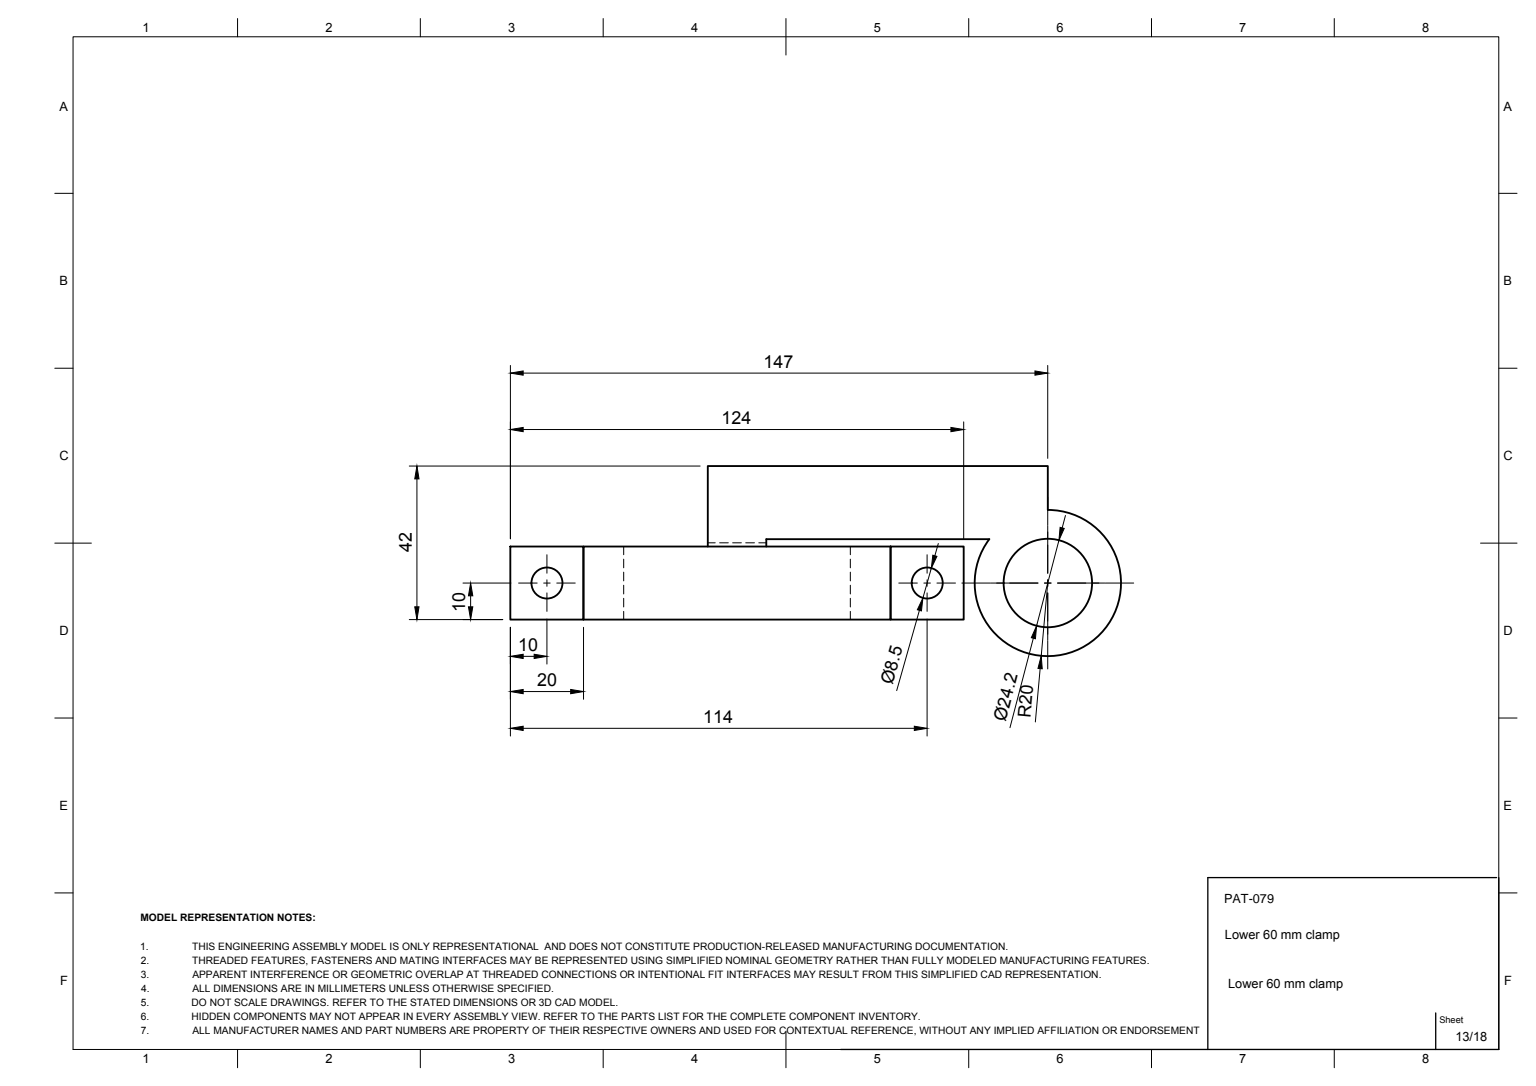
ISO-10303-21;
HEADER;
/* Generated by software containing ST-Developer
 * from STEP Tools, Inc. (www.steptools.com) 
 */

FILE_DESCRIPTION(
/* description */ ('Pipe clamp stand with threaded column'),
/* implementation_level */ '2;1');

FILE_NAME(
/* name */ 'Lower 60 mm clamp.step',
/* time_stamp */ '2026-10-27T10:55:48-07:00',
/* author */ (''),
/* organization */ (''),
/* preprocessor_version */ 'ST-DEVELOPER v20.2',
/* originating_system */ 'Autodesk Translation Framework v15.17.0.0',
/* authorisation */ '');

FILE_SCHEMA (('AUTOMOTIVE_DESIGN { 1 0 10303 214 3 1 1 }'));
ENDSEC;

DATA;
#10=MECHANICAL_DESIGN_GEOMETRIC_PRESENTATION_REPRESENTATION('',(#753,#754,#755),#34433);
#705=SHAPE_REPRESENTATION_RELATIONSHIP('SRR','None',#34547,#727);
#727=ADVANCED_BREP_SHAPE_REPRESENTATION('',(#783,#784,#785),#34415);
#753=STYLED_ITEM('',(#34757),#783);
#754=STYLED_ITEM('',(#34757),#784);
#755=STYLED_ITEM('',(#34757),#785);
#783=MANIFOLD_SOLID_BREP('Body1',#8780);
#784=MANIFOLD_SOLID_BREP('Body2',#8781);
#785=MANIFOLD_SOLID_BREP('Body3',#8782);
#832=FACE_BOUND('',#1857,.T.);
#833=FACE_BOUND('',#1861,.T.);
#834=FACE_BOUND('',#1869,.T.);
#835=FACE_BOUND('',#1872,.T.);
#836=FACE_BOUND('',#1878,.T.);
#837=FACE_BOUND('',#1881,.T.);
#919=PLANE('',#9405);
#920=PLANE('',#9406);
#921=PLANE('',#9408);
#922=PLANE('',#9409);
#923=PLANE('',#9416);
#924=PLANE('',#9417);
#925=PLANE('',#9418);
#926=PLANE('',#9419);
#927=PLANE('',#9420);
#928=PLANE('',#9421);
#929=PLANE('',#9422);
#930=PLANE('',#9423);
#931=PLANE('',#9429);
#932=PLANE('',#9430);
#933=PLANE('',#9431);
#934=PLANE('',#9432);
#935=PLANE('',#9433);
#936=PLANE('',#9434);
#937=PLANE('',#9438);
#938=PLANE('',#9439);
#939=PLANE('',#9440);
#940=PLANE('',#9441);
#941=PLANE('',#9442);
#942=PLANE('',#9443);
#1328=FACE_OUTER_BOUND('',#1848,.T.);
#1329=FACE_OUTER_BOUND('',#1849,.T.);
#1330=FACE_OUTER_BOUND('',#1850,.T.);
#1331=FACE_OUTER_BOUND('',#1851,.T.);
#1332=FACE_OUTER_BOUND('',#1852,.T.);
#1333=FACE_OUTER_BOUND('',#1853,.T.);
#1334=FACE_OUTER_BOUND('',#1854,.T.);
#1335=FACE_OUTER_BOUND('',#1855,.T.);
#1336=FACE_OUTER_BOUND('',#1856,.T.);
#1337=FACE_OUTER_BOUND('',#1858,.T.);
#1338=FACE_OUTER_BOUND('',#1859,.T.);
#1339=FACE_OUTER_BOUND('',#1860,.T.);
#1340=FACE_OUTER_BOUND('',#1862,.T.);
#1341=FACE_OUTER_BOUND('',#1863,.T.);
#1342=FACE_OUTER_BOUND('',#1864,.T.);
#1343=FACE_OUTER_BOUND('',#1865,.T.);
#1344=FACE_OUTER_BOUND('',#1866,.T.);
#1345=FACE_OUTER_BOUND('',#1867,.T.);
#1346=FACE_OUTER_BOUND('',#1868,.T.);
#1347=FACE_OUTER_BOUND('',#1870,.T.);
#1348=FACE_OUTER_BOUND('',#1871,.T.);
#1349=FACE_OUTER_BOUND('',#1873,.T.);
#1350=FACE_OUTER_BOUND('',#1874,.T.);
#1351=FACE_OUTER_BOUND('',#1875,.T.);
#1352=FACE_OUTER_BOUND('',#1876,.T.);
#1353=FACE_OUTER_BOUND('',#1877,.T.);
#1354=FACE_OUTER_BOUND('',#1879,.T.);
#1355=FACE_OUTER_BOUND('',#1880,.T.);
#1356=FACE_OUTER_BOUND('',#1882,.T.);
#1357=FACE_OUTER_BOUND('',#1883,.T.);
#1848=EDGE_LOOP('',(#7055,#7056,#7057,#7058,#7059,#7060,#7061,#7062));
#1849=EDGE_LOOP('',(#7063,#7064,#7065,#7066));
#1850=EDGE_LOOP('',(#7067,#7068,#7069,#7070));
#1851=EDGE_LOOP('',(#7071,#7072,#7073,#7074));
#1852=EDGE_LOOP('',(#7075,#7076,#7077,#7078,#7079,#7080));
#1853=EDGE_LOOP('',(#7081,#7082,#7083,#7084));
#1854=EDGE_LOOP('',(#7085,#7086,#7087,#7088));
#1855=EDGE_LOOP('',(#7089,#7090,#7091,#7092));
#1856=EDGE_LOOP('',(#7093,#7094,#7095,#7096,#7097,#7098,#7099));
#1857=EDGE_LOOP('',(#7100));
#1858=EDGE_LOOP('',(#7101,#7102,#7103,#7104));
#1859=EDGE_LOOP('',(#7105,#7106,#7107,#7108));
#1860=EDGE_LOOP('',(#7109,#7110,#7111,#7112,#7113,#7114,#7115));
#1861=EDGE_LOOP('',(#7116));
#1862=EDGE_LOOP('',(#7117,#7118,#7119,#7120,#7121,#7122));
#1863=EDGE_LOOP('',(#7123,#7124,#7125,#7126));
#1864=EDGE_LOOP('',(#7127,#7128,#7129,#7130,#7131,#7132,#7133,#7134));
#1865=EDGE_LOOP('',(#7135,#7136,#7137,#7138));
#1866=EDGE_LOOP('',(#7139,#7140,#7141,#7142));
#1867=EDGE_LOOP('',(#7143,#7144,#7145,#7146));
#1868=EDGE_LOOP('',(#7147,#7148,#7149,#7150));
#1869=EDGE_LOOP('',(#7151));
#1870=EDGE_LOOP('',(#7152,#7153,#7154,#7155));
#1871=EDGE_LOOP('',(#7156,#7157,#7158,#7159));
#1872=EDGE_LOOP('',(#7160));
#1873=EDGE_LOOP('',(#7161,#7162,#7163,#7164));
#1874=EDGE_LOOP('',(#7165,#7166,#7167,#7168));
#1875=EDGE_LOOP('',(#7169,#7170,#7171,#7172));
#1876=EDGE_LOOP('',(#7173,#7174,#7175,#7176));
#1877=EDGE_LOOP('',(#7177,#7178,#7179,#7180));
#1878=EDGE_LOOP('',(#7181));
#1879=EDGE_LOOP('',(#7182,#7183,#7184,#7185));
#1880=EDGE_LOOP('',(#7186,#7187,#7188,#7189));
#1881=EDGE_LOOP('',(#7190));
#1882=EDGE_LOOP('',(#7191,#7192,#7193,#7194));
#1883=EDGE_LOOP('',(#7195,#7196,#7197,#7198));
#2399=LINE('',#28332,#3016);
#2400=LINE('',#28336,#3017);
#2401=LINE('',#28340,#3018);
#2402=LINE('',#28344,#3019);
#2403=LINE('',#28348,#3020);
#2404=LINE('',#28350,#3021);
#2405=LINE('',#28351,#3022);
#2406=LINE('',#28354,#3023);
#2407=LINE('',#28357,#3024);
#2408=LINE('',#28360,#3025);
#2409=LINE('',#28361,#3026);
#2410=LINE('',#28364,#3027);
#2411=LINE('',#28366,#3028);
#2412=LINE('',#28368,#3029);
#2413=LINE('',#28369,#3030);
#2414=LINE('',#28374,#3031);
#2415=LINE('',#28379,#3032);
#2416=LINE('',#28383,#3033);
#2417=LINE('',#28386,#3034);
#2418=LINE('',#28387,#3035);
#2419=LINE('',#28390,#3036);
#2420=LINE('',#28392,#3037);
#2421=LINE('',#28394,#3038);
#2422=LINE('',#28395,#3039);
#2423=LINE('',#28398,#3040);
#2424=LINE('',#28399,#3041);
#2425=LINE('',#28402,#3042);
#2426=LINE('',#28403,#3043);
#2427=LINE('',#28405,#3044);
#2428=LINE('',#28407,#3045);
#2429=LINE('',#28410,#3046);
#2430=LINE('',#28411,#3047);
#2431=LINE('',#28419,#3048);
#2432=LINE('',#28424,#3049);
#2433=LINE('',#28426,#3050);
#2434=LINE('',#28428,#3051);
#2435=LINE('',#28429,#3052);
#2436=LINE('',#28432,#3053);
#2437=LINE('',#28434,#3054);
#2438=LINE('',#28435,#3055);
#2439=LINE('',#28438,#3056);
#2440=LINE('',#28440,#3057);
#2441=LINE('',#28441,#3058);
#2442=LINE('',#28443,#3059);
#2443=LINE('',#28444,#3060);
#2444=LINE('',#28451,#3061);
#2445=LINE('',#28456,#3062);
#2446=LINE('',#28458,#3063);
#2447=LINE('',#28460,#3064);
#2448=LINE('',#28461,#3065);
#2449=LINE('',#28464,#3066);
#2450=LINE('',#28466,#3067);
#2451=LINE('',#28467,#3068);
#2452=LINE('',#28470,#3069);
#2453=LINE('',#28472,#3070);
#2454=LINE('',#28473,#3071);
#2455=LINE('',#28475,#3072);
#2456=LINE('',#28476,#3073);
#3016=VECTOR('',#10764,1.);
#3017=VECTOR('',#10767,1.);
#3018=VECTOR('',#10770,1.);
#3019=VECTOR('',#10773,1.);
#3020=VECTOR('',#10778,1.);
#3021=VECTOR('',#10779,1.);
#3022=VECTOR('',#10780,1.);
#3023=VECTOR('',#10783,1.);
#3024=VECTOR('',#10786,1.);
#3025=VECTOR('',#10789,1.);
#3026=VECTOR('',#10790,1.);
#3027=VECTOR('',#10793,1.);
#3028=VECTOR('',#10794,1.);
#3029=VECTOR('',#10795,1.);
#3030=VECTOR('',#10796,1.);
#3031=VECTOR('',#10801,1.21);
#3032=VECTOR('',#10806,1.);
#3033=VECTOR('',#10809,1.);
#3034=VECTOR('',#10814,1.);
#3035=VECTOR('',#10815,1.);
#3036=VECTOR('',#10818,1.);
#3037=VECTOR('',#10819,1.);
#3038=VECTOR('',#10820,1.);
#3039=VECTOR('',#10821,1.);
#3040=VECTOR('',#10824,1.);
#3041=VECTOR('',#10825,1.);
#3042=VECTOR('',#10828,1.);
#3043=VECTOR('',#10829,1.);
#3044=VECTOR('',#10832,1.);
#3045=VECTOR('',#10835,1.);
#3046=VECTOR('',#10838,1.);
#3047=VECTOR('',#10839,1.);
#3048=VECTOR('',#10850,0.425);
#3049=VECTOR('',#10855,1.);
#3050=VECTOR('',#10856,1.);
#3051=VECTOR('',#10857,1.);
#3052=VECTOR('',#10858,1.);
#3053=VECTOR('',#10861,1.);
#3054=VECTOR('',#10862,1.);
#3055=VECTOR('',#10863,1.);
#3056=VECTOR('',#10866,1.);
#3057=VECTOR('',#10867,1.);
#3058=VECTOR('',#10868,1.);
#3059=VECTOR('',#10871,1.);
#3060=VECTOR('',#10872,1.);
#3061=VECTOR('',#10881,0.425);
#3062=VECTOR('',#10886,1.);
#3063=VECTOR('',#10887,1.);
#3064=VECTOR('',#10888,1.);
#3065=VECTOR('',#10889,1.);
#3066=VECTOR('',#10892,1.);
#3067=VECTOR('',#10893,1.);
#3068=VECTOR('',#10894,1.);
#3069=VECTOR('',#10897,1.);
#3070=VECTOR('',#10898,1.);
#3071=VECTOR('',#10899,1.);
#3072=VECTOR('',#10902,1.);
#3073=VECTOR('',#10903,1.);
#3374=CIRCLE('',#9401,3.1);
#3375=CIRCLE('',#9402,3.1);
#3376=CIRCLE('',#9403,3.1);
#3377=CIRCLE('',#9404,3.1);
#3378=CIRCLE('',#9407,4.2);
#3379=CIRCLE('',#9411,1.21);
#3380=CIRCLE('',#9412,1.21);
#3381=CIRCLE('',#9414,2.);
#3382=CIRCLE('',#9415,2.);
#3383=CIRCLE('',#9424,4.2);
#3384=CIRCLE('',#9427,0.425);
#3385=CIRCLE('',#9428,0.425);
#3386=CIRCLE('',#9436,0.425);
#3387=CIRCLE('',#9437,0.425);
#3958=VERTEX_POINT('',#28330);
#3959=VERTEX_POINT('',#28331);
#3960=VERTEX_POINT('',#28333);
#3961=VERTEX_POINT('',#28335);
#3962=VERTEX_POINT('',#28337);
#3963=VERTEX_POINT('',#28339);
#3964=VERTEX_POINT('',#28341);
#3965=VERTEX_POINT('',#28343);
#3966=VERTEX_POINT('',#28347);
#3967=VERTEX_POINT('',#28349);
#3968=VERTEX_POINT('',#28353);
#3969=VERTEX_POINT('',#28355);
#3970=VERTEX_POINT('',#28359);
#3971=VERTEX_POINT('',#28363);
#3972=VERTEX_POINT('',#28365);
#3973=VERTEX_POINT('',#28367);
#3974=VERTEX_POINT('',#28371);
#3975=VERTEX_POINT('',#28373);
#3976=VERTEX_POINT('',#28377);
#3977=VERTEX_POINT('',#28378);
#3978=VERTEX_POINT('',#28380);
#3979=VERTEX_POINT('',#28382);
#3980=VERTEX_POINT('',#28389);
#3981=VERTEX_POINT('',#28391);
#3982=VERTEX_POINT('',#28393);
#3983=VERTEX_POINT('',#28397);
#3984=VERTEX_POINT('',#28401);
#3985=VERTEX_POINT('',#28409);
#3986=VERTEX_POINT('',#28416);
#3987=VERTEX_POINT('',#28418);
#3988=VERTEX_POINT('',#28422);
#3989=VERTEX_POINT('',#28423);
#3990=VERTEX_POINT('',#28425);
#3991=VERTEX_POINT('',#28427);
#3992=VERTEX_POINT('',#28431);
#3993=VERTEX_POINT('',#28433);
#3994=VERTEX_POINT('',#28437);
#3995=VERTEX_POINT('',#28439);
#3996=VERTEX_POINT('',#28448);
#3997=VERTEX_POINT('',#28450);
#3998=VERTEX_POINT('',#28454);
#3999=VERTEX_POINT('',#28455);
#4000=VERTEX_POINT('',#28457);
#4001=VERTEX_POINT('',#28459);
#4002=VERTEX_POINT('',#28463);
#4003=VERTEX_POINT('',#28465);
#4004=VERTEX_POINT('',#28469);
#4005=VERTEX_POINT('',#28471);
#5041=EDGE_CURVE('',#3958,#3959,#2399,.T.);
#5042=EDGE_CURVE('',#3958,#3960,#3374,.T.);
#5043=EDGE_CURVE('',#3961,#3960,#2400,.T.);
#5044=EDGE_CURVE('',#3962,#3961,#3375,.T.);
#5045=EDGE_CURVE('',#3963,#3962,#2401,.T.);
#5046=EDGE_CURVE('',#3964,#3963,#3376,.T.);
#5047=EDGE_CURVE('',#3965,#3964,#2402,.T.);
#5048=EDGE_CURVE('',#3959,#3965,#3377,.T.);
#5049=EDGE_CURVE('',#3966,#3958,#2403,.T.);
#5050=EDGE_CURVE('',#3967,#3966,#2404,.T.);
#5051=EDGE_CURVE('',#3960,#3967,#2405,.T.);
#5052=EDGE_CURVE('',#3963,#3968,#2406,.T.);
#5053=EDGE_CURVE('',#3969,#3968,#3378,.T.);
#5054=EDGE_CURVE('',#3969,#3964,#2407,.T.);
#5055=EDGE_CURVE('',#3970,#3962,#2408,.T.);
#5056=EDGE_CURVE('',#3968,#3970,#2409,.T.);
#5057=EDGE_CURVE('',#3967,#3971,#2410,.T.);
#5058=EDGE_CURVE('',#3971,#3972,#2411,.T.);
#5059=EDGE_CURVE('',#3973,#3972,#2412,.T.);
#5060=EDGE_CURVE('',#3961,#3973,#2413,.T.);
#5061=EDGE_CURVE('',#3974,#3974,#3379,.T.);
#5062=EDGE_CURVE('',#3974,#3975,#2414,.T.);
#5063=EDGE_CURVE('',#3975,#3975,#3380,.T.);
#5064=EDGE_CURVE('',#3976,#3977,#2415,.T.);
#5065=EDGE_CURVE('',#3978,#3976,#3381,.T.);
#5066=EDGE_CURVE('',#3979,#3978,#2416,.T.);
#5067=EDGE_CURVE('',#3979,#3977,#3382,.T.);
#5068=EDGE_CURVE('',#3977,#3972,#2417,.T.);
#5069=EDGE_CURVE('',#3971,#3976,#2418,.T.);
#5070=EDGE_CURVE('',#3979,#3980,#2419,.T.);
#5071=EDGE_CURVE('',#3981,#3980,#2420,.T.);
#5072=EDGE_CURVE('',#3982,#3981,#2421,.T.);
#5073=EDGE_CURVE('',#3973,#3982,#2422,.T.);
#5074=EDGE_CURVE('',#3978,#3983,#2423,.T.);
#5075=EDGE_CURVE('',#3980,#3983,#2424,.T.);
#5076=EDGE_CURVE('',#3983,#3984,#2425,.T.);
#5077=EDGE_CURVE('',#3984,#3981,#2426,.T.);
#5078=EDGE_CURVE('',#3966,#3984,#2427,.T.);
#5079=EDGE_CURVE('',#3982,#3959,#2428,.T.);
#5080=EDGE_CURVE('',#3985,#3969,#2429,.T.);
#5081=EDGE_CURVE('',#3965,#3985,#2430,.T.);
#5082=EDGE_CURVE('',#3985,#3970,#3383,.T.);
#5083=EDGE_CURVE('',#3986,#3986,#3384,.T.);
#5084=EDGE_CURVE('',#3986,#3987,#2431,.T.);
#5085=EDGE_CURVE('',#3987,#3987,#3385,.T.);
#5086=EDGE_CURVE('',#3988,#3989,#2432,.T.);
#5087=EDGE_CURVE('',#3988,#3990,#2433,.T.);
#5088=EDGE_CURVE('',#3991,#3990,#2434,.T.);
#5089=EDGE_CURVE('',#3989,#3991,#2435,.T.);
#5090=EDGE_CURVE('',#3989,#3992,#2436,.T.);
#5091=EDGE_CURVE('',#3993,#3991,#2437,.T.);
#5092=EDGE_CURVE('',#3992,#3993,#2438,.T.);
#5093=EDGE_CURVE('',#3992,#3994,#2439,.T.);
#5094=EDGE_CURVE('',#3995,#3993,#2440,.T.);
#5095=EDGE_CURVE('',#3994,#3995,#2441,.T.);
#5096=EDGE_CURVE('',#3994,#3988,#2442,.T.);
#5097=EDGE_CURVE('',#3990,#3995,#2443,.T.);
#5098=EDGE_CURVE('',#3996,#3996,#3386,.T.);
#5099=EDGE_CURVE('',#3996,#3997,#2444,.T.);
#5100=EDGE_CURVE('',#3997,#3997,#3387,.T.);
#5101=EDGE_CURVE('',#3998,#3999,#2445,.T.);
#5102=EDGE_CURVE('',#3998,#4000,#2446,.T.);
#5103=EDGE_CURVE('',#4001,#4000,#2447,.T.);
#5104=EDGE_CURVE('',#3999,#4001,#2448,.T.);
#5105=EDGE_CURVE('',#3999,#4002,#2449,.T.);
#5106=EDGE_CURVE('',#4003,#4001,#2450,.T.);
#5107=EDGE_CURVE('',#4002,#4003,#2451,.T.);
#5108=EDGE_CURVE('',#4002,#4004,#2452,.T.);
#5109=EDGE_CURVE('',#4005,#4003,#2453,.T.);
#5110=EDGE_CURVE('',#4004,#4005,#2454,.T.);
#5111=EDGE_CURVE('',#4004,#3998,#2455,.T.);
#5112=EDGE_CURVE('',#4000,#4005,#2456,.T.);
#7055=ORIENTED_EDGE('',*,*,#5041,.F.);
#7056=ORIENTED_EDGE('',*,*,#5042,.T.);
#7057=ORIENTED_EDGE('',*,*,#5043,.F.);
#7058=ORIENTED_EDGE('',*,*,#5044,.F.);
#7059=ORIENTED_EDGE('',*,*,#5045,.F.);
#7060=ORIENTED_EDGE('',*,*,#5046,.F.);
#7061=ORIENTED_EDGE('',*,*,#5047,.F.);
#7062=ORIENTED_EDGE('',*,*,#5048,.F.);
#7063=ORIENTED_EDGE('',*,*,#5049,.F.);
#7064=ORIENTED_EDGE('',*,*,#5050,.F.);
#7065=ORIENTED_EDGE('',*,*,#5051,.F.);
#7066=ORIENTED_EDGE('',*,*,#5042,.F.);
#7067=ORIENTED_EDGE('',*,*,#5046,.T.);
#7068=ORIENTED_EDGE('',*,*,#5052,.T.);
#7069=ORIENTED_EDGE('',*,*,#5053,.F.);
#7070=ORIENTED_EDGE('',*,*,#5054,.T.);
#7071=ORIENTED_EDGE('',*,*,#5045,.T.);
#7072=ORIENTED_EDGE('',*,*,#5055,.F.);
#7073=ORIENTED_EDGE('',*,*,#5056,.F.);
#7074=ORIENTED_EDGE('',*,*,#5052,.F.);
#7075=ORIENTED_EDGE('',*,*,#5043,.T.);
#7076=ORIENTED_EDGE('',*,*,#5051,.T.);
#7077=ORIENTED_EDGE('',*,*,#5057,.T.);
#7078=ORIENTED_EDGE('',*,*,#5058,.T.);
#7079=ORIENTED_EDGE('',*,*,#5059,.F.);
#7080=ORIENTED_EDGE('',*,*,#5060,.F.);
#7081=ORIENTED_EDGE('',*,*,#5061,.F.);
#7082=ORIENTED_EDGE('',*,*,#5062,.T.);
#7083=ORIENTED_EDGE('',*,*,#5063,.F.);
#7084=ORIENTED_EDGE('',*,*,#5062,.F.);
#7085=ORIENTED_EDGE('',*,*,#5064,.F.);
#7086=ORIENTED_EDGE('',*,*,#5065,.F.);
#7087=ORIENTED_EDGE('',*,*,#5066,.F.);
#7088=ORIENTED_EDGE('',*,*,#5067,.T.);
#7089=ORIENTED_EDGE('',*,*,#5064,.T.);
#7090=ORIENTED_EDGE('',*,*,#5068,.T.);
#7091=ORIENTED_EDGE('',*,*,#5058,.F.);
#7092=ORIENTED_EDGE('',*,*,#5069,.T.);
#7093=ORIENTED_EDGE('',*,*,#5070,.T.);
#7094=ORIENTED_EDGE('',*,*,#5071,.F.);
#7095=ORIENTED_EDGE('',*,*,#5072,.F.);
#7096=ORIENTED_EDGE('',*,*,#5073,.F.);
#7097=ORIENTED_EDGE('',*,*,#5059,.T.);
#7098=ORIENTED_EDGE('',*,*,#5068,.F.);
#7099=ORIENTED_EDGE('',*,*,#5067,.F.);
#7100=ORIENTED_EDGE('',*,*,#5061,.T.);
#7101=ORIENTED_EDGE('',*,*,#5066,.T.);
#7102=ORIENTED_EDGE('',*,*,#5074,.T.);
#7103=ORIENTED_EDGE('',*,*,#5075,.F.);
#7104=ORIENTED_EDGE('',*,*,#5070,.F.);
#7105=ORIENTED_EDGE('',*,*,#5076,.T.);
#7106=ORIENTED_EDGE('',*,*,#5077,.T.);
#7107=ORIENTED_EDGE('',*,*,#5071,.T.);
#7108=ORIENTED_EDGE('',*,*,#5075,.T.);
#7109=ORIENTED_EDGE('',*,*,#5050,.T.);
#7110=ORIENTED_EDGE('',*,*,#5078,.T.);
#7111=ORIENTED_EDGE('',*,*,#5076,.F.);
#7112=ORIENTED_EDGE('',*,*,#5074,.F.);
#7113=ORIENTED_EDGE('',*,*,#5065,.T.);
#7114=ORIENTED_EDGE('',*,*,#5069,.F.);
#7115=ORIENTED_EDGE('',*,*,#5057,.F.);
#7116=ORIENTED_EDGE('',*,*,#5063,.T.);
#7117=ORIENTED_EDGE('',*,*,#5041,.T.);
#7118=ORIENTED_EDGE('',*,*,#5079,.F.);
#7119=ORIENTED_EDGE('',*,*,#5072,.T.);
#7120=ORIENTED_EDGE('',*,*,#5077,.F.);
#7121=ORIENTED_EDGE('',*,*,#5078,.F.);
#7122=ORIENTED_EDGE('',*,*,#5049,.T.);
#7123=ORIENTED_EDGE('',*,*,#5047,.T.);
#7124=ORIENTED_EDGE('',*,*,#5054,.F.);
#7125=ORIENTED_EDGE('',*,*,#5080,.F.);
#7126=ORIENTED_EDGE('',*,*,#5081,.F.);
#7127=ORIENTED_EDGE('',*,*,#5048,.T.);
#7128=ORIENTED_EDGE('',*,*,#5081,.T.);
#7129=ORIENTED_EDGE('',*,*,#5082,.T.);
#7130=ORIENTED_EDGE('',*,*,#5055,.T.);
#7131=ORIENTED_EDGE('',*,*,#5044,.T.);
#7132=ORIENTED_EDGE('',*,*,#5060,.T.);
#7133=ORIENTED_EDGE('',*,*,#5073,.T.);
#7134=ORIENTED_EDGE('',*,*,#5079,.T.);
#7135=ORIENTED_EDGE('',*,*,#5056,.T.);
#7136=ORIENTED_EDGE('',*,*,#5082,.F.);
#7137=ORIENTED_EDGE('',*,*,#5080,.T.);
#7138=ORIENTED_EDGE('',*,*,#5053,.T.);
#7139=ORIENTED_EDGE('',*,*,#5083,.F.);
#7140=ORIENTED_EDGE('',*,*,#5084,.T.);
#7141=ORIENTED_EDGE('',*,*,#5085,.F.);
#7142=ORIENTED_EDGE('',*,*,#5084,.F.);
#7143=ORIENTED_EDGE('',*,*,#5086,.F.);
#7144=ORIENTED_EDGE('',*,*,#5087,.T.);
#7145=ORIENTED_EDGE('',*,*,#5088,.F.);
#7146=ORIENTED_EDGE('',*,*,#5089,.F.);
#7147=ORIENTED_EDGE('',*,*,#5090,.F.);
#7148=ORIENTED_EDGE('',*,*,#5089,.T.);
#7149=ORIENTED_EDGE('',*,*,#5091,.F.);
#7150=ORIENTED_EDGE('',*,*,#5092,.F.);
#7151=ORIENTED_EDGE('',*,*,#5083,.T.);
#7152=ORIENTED_EDGE('',*,*,#5093,.F.);
#7153=ORIENTED_EDGE('',*,*,#5092,.T.);
#7154=ORIENTED_EDGE('',*,*,#5094,.F.);
#7155=ORIENTED_EDGE('',*,*,#5095,.F.);
#7156=ORIENTED_EDGE('',*,*,#5096,.F.);
#7157=ORIENTED_EDGE('',*,*,#5095,.T.);
#7158=ORIENTED_EDGE('',*,*,#5097,.F.);
#7159=ORIENTED_EDGE('',*,*,#5087,.F.);
#7160=ORIENTED_EDGE('',*,*,#5085,.T.);
#7161=ORIENTED_EDGE('',*,*,#5097,.T.);
#7162=ORIENTED_EDGE('',*,*,#5094,.T.);
#7163=ORIENTED_EDGE('',*,*,#5091,.T.);
#7164=ORIENTED_EDGE('',*,*,#5088,.T.);
#7165=ORIENTED_EDGE('',*,*,#5096,.T.);
#7166=ORIENTED_EDGE('',*,*,#5086,.T.);
#7167=ORIENTED_EDGE('',*,*,#5090,.T.);
#7168=ORIENTED_EDGE('',*,*,#5093,.T.);
#7169=ORIENTED_EDGE('',*,*,#5098,.F.);
#7170=ORIENTED_EDGE('',*,*,#5099,.T.);
#7171=ORIENTED_EDGE('',*,*,#5100,.F.);
#7172=ORIENTED_EDGE('',*,*,#5099,.F.);
#7173=ORIENTED_EDGE('',*,*,#5101,.F.);
#7174=ORIENTED_EDGE('',*,*,#5102,.T.);
#7175=ORIENTED_EDGE('',*,*,#5103,.F.);
#7176=ORIENTED_EDGE('',*,*,#5104,.F.);
#7177=ORIENTED_EDGE('',*,*,#5105,.F.);
#7178=ORIENTED_EDGE('',*,*,#5104,.T.);
#7179=ORIENTED_EDGE('',*,*,#5106,.F.);
#7180=ORIENTED_EDGE('',*,*,#5107,.F.);
#7181=ORIENTED_EDGE('',*,*,#5098,.T.);
#7182=ORIENTED_EDGE('',*,*,#5108,.F.);
#7183=ORIENTED_EDGE('',*,*,#5107,.T.);
#7184=ORIENTED_EDGE('',*,*,#5109,.F.);
#7185=ORIENTED_EDGE('',*,*,#5110,.F.);
#7186=ORIENTED_EDGE('',*,*,#5111,.F.);
#7187=ORIENTED_EDGE('',*,*,#5110,.T.);
#7188=ORIENTED_EDGE('',*,*,#5112,.F.);
#7189=ORIENTED_EDGE('',*,*,#5102,.F.);
#7190=ORIENTED_EDGE('',*,*,#5100,.T.);
#7191=ORIENTED_EDGE('',*,*,#5112,.T.);
#7192=ORIENTED_EDGE('',*,*,#5109,.T.);
#7193=ORIENTED_EDGE('',*,*,#5106,.T.);
#7194=ORIENTED_EDGE('',*,*,#5103,.T.);
#7195=ORIENTED_EDGE('',*,*,#5111,.T.);
#7196=ORIENTED_EDGE('',*,*,#5101,.T.);
#7197=ORIENTED_EDGE('',*,*,#5105,.T.);
#7198=ORIENTED_EDGE('',*,*,#5108,.T.);
#8219=CYLINDRICAL_SURFACE('',#9400,3.1);
#8220=CYLINDRICAL_SURFACE('',#9410,1.21);
#8221=CYLINDRICAL_SURFACE('',#9413,2.);
#8222=CYLINDRICAL_SURFACE('',#9425,4.2);
#8223=CYLINDRICAL_SURFACE('',#9426,0.425);
#8224=CYLINDRICAL_SURFACE('',#9435,0.425);
#8565=ADVANCED_FACE('',(#1328),#8219,.F.);
#8566=ADVANCED_FACE('',(#1329),#919,.F.);
#8567=ADVANCED_FACE('',(#1330),#920,.F.);
#8568=ADVANCED_FACE('',(#1331),#921,.F.);
#8569=ADVANCED_FACE('',(#1332),#922,.T.);
#8570=ADVANCED_FACE('',(#1333),#8220,.F.);
#8571=ADVANCED_FACE('',(#1334),#8221,.T.);
#8572=ADVANCED_FACE('',(#1335),#923,.F.);
#8573=ADVANCED_FACE('',(#1336,#832),#924,.T.);
#8574=ADVANCED_FACE('',(#1337),#925,.T.);
#8575=ADVANCED_FACE('',(#1338),#926,.T.);
#8576=ADVANCED_FACE('',(#1339,#833),#927,.T.);
#8577=ADVANCED_FACE('',(#1340),#928,.T.);
#8578=ADVANCED_FACE('',(#1341),#929,.F.);
#8579=ADVANCED_FACE('',(#1342),#930,.T.);
#8580=ADVANCED_FACE('',(#1343),#8222,.T.);
#8581=ADVANCED_FACE('',(#1344),#8223,.F.);
#8582=ADVANCED_FACE('',(#1345),#931,.T.);
#8583=ADVANCED_FACE('',(#1346,#834),#932,.T.);
#8584=ADVANCED_FACE('',(#1347),#933,.T.);
#8585=ADVANCED_FACE('',(#1348,#835),#934,.T.);
#8586=ADVANCED_FACE('',(#1349),#935,.T.);
#8587=ADVANCED_FACE('',(#1350),#936,.F.);
#8588=ADVANCED_FACE('',(#1351),#8224,.F.);
#8589=ADVANCED_FACE('',(#1352),#937,.T.);
#8590=ADVANCED_FACE('',(#1353,#836),#938,.T.);
#8591=ADVANCED_FACE('',(#1354),#939,.T.);
#8592=ADVANCED_FACE('',(#1355,#837),#940,.T.);
#8593=ADVANCED_FACE('',(#1356),#941,.T.);
#8594=ADVANCED_FACE('',(#1357),#942,.F.);
#8780=CLOSED_SHELL('',(#8565,#8566,#8567,#8568,#8569,#8570,#8571,#8572,
#8573,#8574,#8575,#8576,#8577,#8578,#8579,#8580));
#8781=CLOSED_SHELL('',(#8581,#8582,#8583,#8584,#8585,#8586,#8587));
#8782=CLOSED_SHELL('',(#8588,#8589,#8590,#8591,#8592,#8593,#8594));
#9399=AXIS2_PLACEMENT_3D('',#28328,#10760,#10761);
#9400=AXIS2_PLACEMENT_3D('',#28329,#10762,#10763);
#9401=AXIS2_PLACEMENT_3D('',#28334,#10765,#10766);
#9402=AXIS2_PLACEMENT_3D('',#28338,#10768,#10769);
#9403=AXIS2_PLACEMENT_3D('',#28342,#10771,#10772);
#9404=AXIS2_PLACEMENT_3D('',#28345,#10774,#10775);
#9405=AXIS2_PLACEMENT_3D('',#28346,#10776,#10777);
#9406=AXIS2_PLACEMENT_3D('',#28352,#10781,#10782);
#9407=AXIS2_PLACEMENT_3D('',#28356,#10784,#10785);
#9408=AXIS2_PLACEMENT_3D('',#28358,#10787,#10788);
#9409=AXIS2_PLACEMENT_3D('',#28362,#10791,#10792);
#9410=AXIS2_PLACEMENT_3D('',#28370,#10797,#10798);
#9411=AXIS2_PLACEMENT_3D('',#28372,#10799,#10800);
#9412=AXIS2_PLACEMENT_3D('',#28375,#10802,#10803);
#9413=AXIS2_PLACEMENT_3D('',#28376,#10804,#10805);
#9414=AXIS2_PLACEMENT_3D('',#28381,#10807,#10808);
#9415=AXIS2_PLACEMENT_3D('',#28384,#10810,#10811);
#9416=AXIS2_PLACEMENT_3D('',#28385,#10812,#10813);
#9417=AXIS2_PLACEMENT_3D('',#28388,#10816,#10817);
#9418=AXIS2_PLACEMENT_3D('',#28396,#10822,#10823);
#9419=AXIS2_PLACEMENT_3D('',#28400,#10826,#10827);
#9420=AXIS2_PLACEMENT_3D('',#28404,#10830,#10831);
#9421=AXIS2_PLACEMENT_3D('',#28406,#10833,#10834);
#9422=AXIS2_PLACEMENT_3D('',#28408,#10836,#10837);
#9423=AXIS2_PLACEMENT_3D('',#28412,#10840,#10841);
#9424=AXIS2_PLACEMENT_3D('',#28413,#10842,#10843);
#9425=AXIS2_PLACEMENT_3D('',#28414,#10844,#10845);
#9426=AXIS2_PLACEMENT_3D('',#28415,#10846,#10847);
#9427=AXIS2_PLACEMENT_3D('',#28417,#10848,#10849);
#9428=AXIS2_PLACEMENT_3D('',#28420,#10851,#10852);
#9429=AXIS2_PLACEMENT_3D('',#28421,#10853,#10854);
#9430=AXIS2_PLACEMENT_3D('',#28430,#10859,#10860);
#9431=AXIS2_PLACEMENT_3D('',#28436,#10864,#10865);
#9432=AXIS2_PLACEMENT_3D('',#28442,#10869,#10870);
#9433=AXIS2_PLACEMENT_3D('',#28445,#10873,#10874);
#9434=AXIS2_PLACEMENT_3D('',#28446,#10875,#10876);
#9435=AXIS2_PLACEMENT_3D('',#28447,#10877,#10878);
#9436=AXIS2_PLACEMENT_3D('',#28449,#10879,#10880);
#9437=AXIS2_PLACEMENT_3D('',#28452,#10882,#10883);
#9438=AXIS2_PLACEMENT_3D('',#28453,#10884,#10885);
#9439=AXIS2_PLACEMENT_3D('',#28462,#10890,#10891);
#9440=AXIS2_PLACEMENT_3D('',#28468,#10895,#10896);
#9441=AXIS2_PLACEMENT_3D('',#28474,#10900,#10901);
#9442=AXIS2_PLACEMENT_3D('',#28477,#10904,#10905);
#9443=AXIS2_PLACEMENT_3D('',#28478,#10906,#10907);
#10760=DIRECTION('axis',(0.,0.,1.));
#10761=DIRECTION('refdir',(1.,0.,0.));
#10762=DIRECTION('center_axis',(0.,1.,0.));
#10763=DIRECTION('ref_axis',(1.,0.,0.));
#10764=DIRECTION('',(0.,-1.,0.));
#10765=DIRECTION('center_axis',(0.,1.,0.));
#10766=DIRECTION('ref_axis',(1.,0.,0.));
#10767=DIRECTION('',(0.,1.,0.));
#10768=DIRECTION('center_axis',(0.,-1.,0.));
#10769=DIRECTION('ref_axis',(1.,0.,0.));
#10770=DIRECTION('',(0.,1.,0.));
#10771=DIRECTION('center_axis',(0.,1.,0.));
#10772=DIRECTION('ref_axis',(1.,0.,0.));
#10773=DIRECTION('',(0.,-1.,0.));
#10774=DIRECTION('center_axis',(0.,-1.,0.));
#10775=DIRECTION('ref_axis',(1.,0.,0.));
#10776=DIRECTION('center_axis',(0.,1.,0.));
#10777=DIRECTION('ref_axis',(1.,0.,0.));
#10778=DIRECTION('',(0.,0.,-1.));
#10779=DIRECTION('',(1.,0.,0.));
#10780=DIRECTION('',(0.,0.,1.));
#10781=DIRECTION('center_axis',(0.,1.,0.));
#10782=DIRECTION('ref_axis',(1.,0.,0.));
#10783=DIRECTION('',(-1.,0.,0.));
#10784=DIRECTION('center_axis',(0.,1.,0.));
#10785=DIRECTION('ref_axis',(1.,0.,0.));
#10786=DIRECTION('',(-1.,0.,0.));
#10787=DIRECTION('center_axis',(0.,0.,-1.));
#10788=DIRECTION('ref_axis',(-1.,0.,0.));
#10789=DIRECTION('',(1.,0.,0.));
#10790=DIRECTION('',(0.,1.,0.));
#10791=DIRECTION('center_axis',(-1.,0.,0.));
#10792=DIRECTION('ref_axis',(0.,0.,1.));
#10793=DIRECTION('',(0.,1.,0.));
#10794=DIRECTION('',(0.,0.,-1.));
#10795=DIRECTION('',(0.,1.,0.));
#10796=DIRECTION('',(0.,0.,-1.));
#10797=DIRECTION('center_axis',(0.,0.,1.));
#10798=DIRECTION('ref_axis',(1.,0.,0.));
#10799=DIRECTION('center_axis',(0.,0.,1.));
#10800=DIRECTION('ref_axis',(1.,0.,0.));
#10801=DIRECTION('',(0.,0.,1.));
#10802=DIRECTION('center_axis',(0.,0.,-1.));
#10803=DIRECTION('ref_axis',(1.,0.,0.));
#10804=DIRECTION('center_axis',(0.,0.,1.));
#10805=DIRECTION('ref_axis',(-0.447213595499958,-0.894427190999916,0.));
#10806=DIRECTION('',(0.,0.,-1.));
#10807=DIRECTION('center_axis',(0.,0.,1.));
#10808=DIRECTION('ref_axis',(1.,0.,0.));
#10809=DIRECTION('',(0.,0.,1.));
#10810=DIRECTION('center_axis',(0.,0.,1.));
#10811=DIRECTION('ref_axis',(1.,0.,0.));
#10812=DIRECTION('center_axis',(0.,1.,0.));
#10813=DIRECTION('ref_axis',(1.,0.,0.));
#10814=DIRECTION('',(1.,0.,0.));
#10815=DIRECTION('',(-1.,0.,0.));
#10816=DIRECTION('center_axis',(0.,0.,-1.));
#10817=DIRECTION('ref_axis',(-1.,0.,0.));
#10818=DIRECTION('',(0.,1.,0.));
#10819=DIRECTION('',(-1.,0.,0.));
#10820=DIRECTION('',(0.,1.,0.));
#10821=DIRECTION('',(1.,0.,0.));
#10822=DIRECTION('center_axis',(-1.,0.,0.));
#10823=DIRECTION('ref_axis',(0.,0.,1.));
#10824=DIRECTION('',(0.,1.,0.));
#10825=DIRECTION('',(0.,0.,1.));
#10826=DIRECTION('center_axis',(0.,1.,0.));
#10827=DIRECTION('ref_axis',(0.,0.,1.));
#10828=DIRECTION('',(1.,0.,0.));
#10829=DIRECTION('',(0.,0.,-1.));
#10830=DIRECTION('center_axis',(0.,0.,1.));
#10831=DIRECTION('ref_axis',(1.,0.,0.));
#10832=DIRECTION('',(0.,1.,0.));
#10833=DIRECTION('center_axis',(1.,0.,0.));
#10834=DIRECTION('ref_axis',(0.,0.,-1.));
#10835=DIRECTION('',(0.,0.,1.));
#10836=DIRECTION('center_axis',(0.,0.,-1.));
#10837=DIRECTION('ref_axis',(-1.,0.,0.));
#10838=DIRECTION('',(0.,-1.,0.));
#10839=DIRECTION('',(1.,0.,0.));
#10840=DIRECTION('center_axis',(0.,1.,0.));
#10841=DIRECTION('ref_axis',(1.,0.,0.));
#10842=DIRECTION('center_axis',(0.,1.,0.));
#10843=DIRECTION('ref_axis',(1.,0.,0.));
#10844=DIRECTION('center_axis',(0.,1.,0.));
#10845=DIRECTION('ref_axis',(1.,0.,0.));
#10846=DIRECTION('center_axis',(0.,0.,1.));
#10847=DIRECTION('ref_axis',(1.,0.,0.));
#10848=DIRECTION('center_axis',(0.,0.,1.));
#10849=DIRECTION('ref_axis',(1.,0.,0.));
#10850=DIRECTION('',(0.,0.,1.));
#10851=DIRECTION('center_axis',(0.,0.,-1.));
#10852=DIRECTION('ref_axis',(1.,0.,0.));
#10853=DIRECTION('center_axis',(-1.,0.,0.));
#10854=DIRECTION('ref_axis',(0.,0.,1.));
#10855=DIRECTION('',(0.,0.,-1.));
#10856=DIRECTION('',(0.,1.,0.));
#10857=DIRECTION('',(0.,0.,1.));
#10858=DIRECTION('',(0.,1.,0.));
#10859=DIRECTION('center_axis',(0.,0.,-1.));
#10860=DIRECTION('ref_axis',(-1.,0.,0.));
#10861=DIRECTION('',(1.,0.,0.));
#10862=DIRECTION('',(-1.,0.,0.));
#10863=DIRECTION('',(0.,1.,0.));
#10864=DIRECTION('center_axis',(1.,0.,0.));
#10865=DIRECTION('ref_axis',(0.,0.,-1.));
#10866=DIRECTION('',(0.,0.,1.));
#10867=DIRECTION('',(0.,0.,-1.));
#10868=DIRECTION('',(0.,1.,0.));
#10869=DIRECTION('center_axis',(0.,0.,1.));
#10870=DIRECTION('ref_axis',(1.,0.,0.));
#10871=DIRECTION('',(-1.,0.,0.));
#10872=DIRECTION('',(1.,0.,0.));
#10873=DIRECTION('center_axis',(0.,1.,0.));
#10874=DIRECTION('ref_axis',(0.,0.,1.));
#10875=DIRECTION('center_axis',(0.,1.,0.));
#10876=DIRECTION('ref_axis',(1.,0.,0.));
#10877=DIRECTION('center_axis',(0.,0.,1.));
#10878=DIRECTION('ref_axis',(1.,0.,0.));
#10879=DIRECTION('center_axis',(0.,0.,1.));
#10880=DIRECTION('ref_axis',(1.,0.,0.));
#10881=DIRECTION('',(0.,0.,1.));
#10882=DIRECTION('center_axis',(0.,0.,-1.));
#10883=DIRECTION('ref_axis',(1.,0.,0.));
#10884=DIRECTION('center_axis',(-1.,0.,0.));
#10885=DIRECTION('ref_axis',(0.,0.,1.));
#10886=DIRECTION('',(0.,0.,-1.));
#10887=DIRECTION('',(0.,1.,0.));
#10888=DIRECTION('',(0.,0.,1.));
#10889=DIRECTION('',(0.,1.,0.));
#10890=DIRECTION('center_axis',(0.,0.,-1.));
#10891=DIRECTION('ref_axis',(-1.,0.,0.));
#10892=DIRECTION('',(1.,0.,0.));
#10893=DIRECTION('',(-1.,0.,0.));
#10894=DIRECTION('',(0.,1.,0.));
#10895=DIRECTION('center_axis',(1.,0.,0.));
#10896=DIRECTION('ref_axis',(0.,0.,-1.));
#10897=DIRECTION('',(0.,0.,1.));
#10898=DIRECTION('',(0.,0.,-1.));
#10899=DIRECTION('',(0.,1.,0.));
#10900=DIRECTION('center_axis',(0.,0.,1.));
#10901=DIRECTION('ref_axis',(1.,0.,0.));
#10902=DIRECTION('',(-1.,0.,0.));
#10903=DIRECTION('',(1.,0.,0.));
#10904=DIRECTION('center_axis',(0.,1.,0.));
#10905=DIRECTION('ref_axis',(0.,0.,1.));
#10906=DIRECTION('center_axis',(0.,1.,0.));
#10907=DIRECTION('ref_axis',(1.,0.,0.));
#28328=CARTESIAN_POINT('',(0.,0.,0.));
#28329=CARTESIAN_POINT('Origin',(0.,-1.1,28.));
#28330=CARTESIAN_POINT('',(0.8,1.1,25.0050041736256));
#28331=CARTESIAN_POINT('',(0.8,1.,25.0050041736256));
#28332=CARTESIAN_POINT('',(0.8,-1.1,25.0050041736256));
#28333=CARTESIAN_POINT('',(-0.8,1.1,25.0050041736256));
#28334=CARTESIAN_POINT('Origin',(0.,1.1,28.));
#28335=CARTESIAN_POINT('',(-0.8,1.,25.0050041736256));
#28336=CARTESIAN_POINT('',(-0.8,-1.1,25.0050041736256));
#28337=CARTESIAN_POINT('',(-3.09989919190931,1.,27.975));
#28338=CARTESIAN_POINT('Origin',(0.,1.,28.));
#28339=CARTESIAN_POINT('',(-3.09989919190931,-1.,27.975));
#28340=CARTESIAN_POINT('',(-3.09989919190931,-1.1,27.975));
#28341=CARTESIAN_POINT('',(3.09989919190931,-1.,27.975));
#28342=CARTESIAN_POINT('Origin',(0.,-1.,28.));
#28343=CARTESIAN_POINT('',(3.09989919190931,1.,27.975));
#28344=CARTESIAN_POINT('',(3.09989919190931,-1.1,27.975));
#28345=CARTESIAN_POINT('Origin',(0.,1.,28.));
#28346=CARTESIAN_POINT('Origin',(0.,1.1,28.));
#28347=CARTESIAN_POINT('',(0.8,1.1,25.2));
#28348=CARTESIAN_POINT('',(0.8,1.1,26.6));
#28349=CARTESIAN_POINT('',(-0.8,1.1,25.2));
#28350=CARTESIAN_POINT('',(-0.4,1.1,25.2));
#28351=CARTESIAN_POINT('',(-0.8,1.1,26.));
#28352=CARTESIAN_POINT('Origin',(0.,-1.,28.));
#28353=CARTESIAN_POINT('',(-4.19992559457903,-1.,27.975));
#28354=CARTESIAN_POINT('',(4.2,-1.,27.975));
#28355=CARTESIAN_POINT('',(4.19992559457903,-1.,27.975));
#28356=CARTESIAN_POINT('Origin',(0.,-1.,28.));
#28357=CARTESIAN_POINT('',(4.2,-1.,27.975));
#28358=CARTESIAN_POINT('Origin',(8.4,-1.1,27.975));
#28359=CARTESIAN_POINT('',(-4.19992559457903,1.,27.975));
#28360=CARTESIAN_POINT('',(4.2,1.,27.975));
#28361=CARTESIAN_POINT('',(-4.19992559457903,-1.,27.975));
#28362=CARTESIAN_POINT('Origin',(-0.8,-1.,24.));
#28363=CARTESIAN_POINT('',(-0.8,1.2,25.2));
#28364=CARTESIAN_POINT('',(-0.8,-1.,25.2));
#28365=CARTESIAN_POINT('',(-0.8,1.2,24.));
#28366=CARTESIAN_POINT('',(-0.8,1.2,24.3));
#28367=CARTESIAN_POINT('',(-0.8,1.,24.));
#28368=CARTESIAN_POINT('',(-0.8,-1.,24.));
#28369=CARTESIAN_POINT('',(-0.8,1.,26.));
#28370=CARTESIAN_POINT('Origin',(-8.5,0.,23.9));
#28371=CARTESIAN_POINT('',(-9.71,-1.4818226269683E-16,24.));
#28372=CARTESIAN_POINT('Origin',(-8.5,0.,24.));
#28373=CARTESIAN_POINT('',(-9.71,1.4818226269683E-16,25.2));
#28374=CARTESIAN_POINT('',(-9.71,-1.4818226269683E-16,23.9));
#28375=CARTESIAN_POINT('Origin',(-8.5,0.,25.2));
#28376=CARTESIAN_POINT('Origin',(-8.5,0.,24.));
#28377=CARTESIAN_POINT('',(-6.9,1.2,25.2));
#28378=CARTESIAN_POINT('',(-6.9,1.2,24.));
#28379=CARTESIAN_POINT('',(-6.9,1.2,24.));
#28380=CARTESIAN_POINT('',(-8.5,2.,25.2));
#28381=CARTESIAN_POINT('Origin',(-8.5,0.,25.2));
#28382=CARTESIAN_POINT('',(-8.5,2.,24.));
#28383=CARTESIAN_POINT('',(-8.5,2.,24.));
#28384=CARTESIAN_POINT('Origin',(-8.5,0.,24.));
#28385=CARTESIAN_POINT('Origin',(-4.25,1.2,24.6));
#28386=CARTESIAN_POINT('',(-8.5,1.2,24.));
#28387=CARTESIAN_POINT('',(0.,1.2,25.2));
#28388=CARTESIAN_POINT('Origin',(0.8,-1.,24.));
#28389=CARTESIAN_POINT('',(-8.5,3.2,24.));
#28390=CARTESIAN_POINT('',(-8.5,1.2,24.));
#28391=CARTESIAN_POINT('',(0.8,3.2,24.));
#28392=CARTESIAN_POINT('',(-0.8,3.2,24.));
#28393=CARTESIAN_POINT('',(0.8,1.,24.));
#28394=CARTESIAN_POINT('',(0.8,-1.,24.));
#28395=CARTESIAN_POINT('',(0.4,1.,24.));
#28396=CARTESIAN_POINT('Origin',(-8.5,1.2,24.));
#28397=CARTESIAN_POINT('',(-8.5,3.2,25.2));
#28398=CARTESIAN_POINT('',(-8.5,1.2,25.2));
#28399=CARTESIAN_POINT('',(-8.5,3.2,25.2));
#28400=CARTESIAN_POINT('Origin',(0.,3.2,24.6));
#28401=CARTESIAN_POINT('',(0.8,3.2,25.2));
#28402=CARTESIAN_POINT('',(0.,3.2,25.2));
#28403=CARTESIAN_POINT('',(0.8,3.2,24.));
#28404=CARTESIAN_POINT('Origin',(-0.8,-1.,25.2));
#28405=CARTESIAN_POINT('',(0.8,-1.,25.2));
#28406=CARTESIAN_POINT('Origin',(0.8,-1.,25.2));
#28407=CARTESIAN_POINT('',(0.8,1.,26.6));
#28408=CARTESIAN_POINT('Origin',(8.4,-1.1,27.975));
#28409=CARTESIAN_POINT('',(4.19992559457903,1.,27.975));
#28410=CARTESIAN_POINT('',(4.19992559457903,-1.,27.975));
#28411=CARTESIAN_POINT('',(4.2,1.,27.975));
#28412=CARTESIAN_POINT('Origin',(0.,1.,28.));
#28413=CARTESIAN_POINT('Origin',(0.,1.,28.));
#28414=CARTESIAN_POINT('Origin',(0.,-1.,28.));
#28415=CARTESIAN_POINT('Origin',(-5.2,0.,26.7));
#28416=CARTESIAN_POINT('',(-5.625,-5.20474889637625E-17,26.8));
#28417=CARTESIAN_POINT('Origin',(-5.2,0.,26.8));
#28418=CARTESIAN_POINT('',(-5.625,5.20474889637625E-17,27.975));
#28419=CARTESIAN_POINT('',(-5.625,-5.20474889637625E-17,26.7));
#28420=CARTESIAN_POINT('Origin',(-5.2,0.,27.975));
#28421=CARTESIAN_POINT('Origin',(-6.2,-1.,26.8));
#28422=CARTESIAN_POINT('',(-6.2,-1.,27.975));
#28423=CARTESIAN_POINT('',(-6.2,-1.,26.8));
#28424=CARTESIAN_POINT('',(-6.2,-1.,27.975));
#28425=CARTESIAN_POINT('',(-6.2,1.,27.975));
#28426=CARTESIAN_POINT('',(-6.2,-1.,27.975));
#28427=CARTESIAN_POINT('',(-6.2,1.,26.8));
#28428=CARTESIAN_POINT('',(-6.2,1.,27.975));
#28429=CARTESIAN_POINT('',(-6.2,-1.,26.8));
#28430=CARTESIAN_POINT('Origin',(-4.2,-1.,26.8));
#28431=CARTESIAN_POINT('',(-4.2,-1.,26.8));
#28432=CARTESIAN_POINT('',(-6.2,-1.,26.8));
#28433=CARTESIAN_POINT('',(-4.2,1.,26.8));
#28434=CARTESIAN_POINT('',(-6.2,1.,26.8));
#28435=CARTESIAN_POINT('',(-4.2,-1.,26.8));
#28436=CARTESIAN_POINT('Origin',(-4.2,-1.,27.975));
#28437=CARTESIAN_POINT('',(-4.2,-1.,27.975));
#28438=CARTESIAN_POINT('',(-4.2,-1.,26.8));
#28439=CARTESIAN_POINT('',(-4.2,1.,27.975));
#28440=CARTESIAN_POINT('',(-4.2,1.,26.8));
#28441=CARTESIAN_POINT('',(-4.2,-1.,27.975));
#28442=CARTESIAN_POINT('Origin',(-6.2,-1.,27.975));
#28443=CARTESIAN_POINT('',(-4.2,-1.,27.975));
#28444=CARTESIAN_POINT('',(-4.2,1.,27.975));
#28445=CARTESIAN_POINT('Origin',(-5.2,1.,27.3875));
#28446=CARTESIAN_POINT('Origin',(-5.2,-1.,27.3875));
#28447=CARTESIAN_POINT('Origin',(5.2,0.,26.7));
#28448=CARTESIAN_POINT('',(4.775,-5.20474889637625E-17,26.8));
#28449=CARTESIAN_POINT('Origin',(5.2,0.,26.8));
#28450=CARTESIAN_POINT('',(4.775,5.20474889637625E-17,27.975));
#28451=CARTESIAN_POINT('',(4.775,-5.20474889637625E-17,26.7));
#28452=CARTESIAN_POINT('Origin',(5.2,0.,27.975));
#28453=CARTESIAN_POINT('Origin',(4.2,-1.,26.8));
#28454=CARTESIAN_POINT('',(4.2,-1.,27.975));
#28455=CARTESIAN_POINT('',(4.2,-1.,26.8));
#28456=CARTESIAN_POINT('',(4.2,-1.,27.975));
#28457=CARTESIAN_POINT('',(4.2,1.,27.975));
#28458=CARTESIAN_POINT('',(4.2,-1.,27.975));
#28459=CARTESIAN_POINT('',(4.2,1.,26.8));
#28460=CARTESIAN_POINT('',(4.2,1.,27.975));
#28461=CARTESIAN_POINT('',(4.2,-1.,26.8));
#28462=CARTESIAN_POINT('Origin',(6.2,-1.,26.8));
#28463=CARTESIAN_POINT('',(6.2,-1.,26.8));
#28464=CARTESIAN_POINT('',(4.2,-1.,26.8));
#28465=CARTESIAN_POINT('',(6.2,1.,26.8));
#28466=CARTESIAN_POINT('',(4.2,1.,26.8));
#28467=CARTESIAN_POINT('',(6.2,-1.,26.8));
#28468=CARTESIAN_POINT('Origin',(6.2,-1.,27.975));
#28469=CARTESIAN_POINT('',(6.2,-1.,27.975));
#28470=CARTESIAN_POINT('',(6.2,-1.,26.8));
#28471=CARTESIAN_POINT('',(6.2,1.,27.975));
#28472=CARTESIAN_POINT('',(6.2,1.,26.8));
#28473=CARTESIAN_POINT('',(6.2,-1.,27.975));
#28474=CARTESIAN_POINT('Origin',(4.2,-1.,27.975));
#28475=CARTESIAN_POINT('',(6.2,-1.,27.975));
#28476=CARTESIAN_POINT('',(6.2,1.,27.975));
#28477=CARTESIAN_POINT('Origin',(5.2,1.,27.3875));
#28478=CARTESIAN_POINT('Origin',(5.2,-1.,27.3875));
#34386=UNCERTAINTY_MEASURE_WITH_UNIT(LENGTH_MEASURE(0.001),#34434,
'DISTANCE_ACCURACY_VALUE',
'Maximum model space distance between geometric entities at asserted c
onnectivities');
#34404=UNCERTAINTY_MEASURE_WITH_UNIT(LENGTH_MEASURE(0.001),#34434,
'DISTANCE_ACCURACY_VALUE',
'Maximum model space distance between geometric entities at asserted c
onnectivities');
#34415=(
GEOMETRIC_REPRESENTATION_CONTEXT(3)
GLOBAL_UNCERTAINTY_ASSIGNED_CONTEXT((#34386))
GLOBAL_UNIT_ASSIGNED_CONTEXT((#34434,#34436,#34437))
REPRESENTATION_CONTEXT('','3D')
);
#34433=(
GEOMETRIC_REPRESENTATION_CONTEXT(3)
GLOBAL_UNCERTAINTY_ASSIGNED_CONTEXT((#34404))
GLOBAL_UNIT_ASSIGNED_CONTEXT((#34434,#34436,#34437))
REPRESENTATION_CONTEXT('','3D')
);
#34434=(
LENGTH_UNIT()
NAMED_UNIT(*)
SI_UNIT(.CENTI.,.METRE.)
);
#34436=(
NAMED_UNIT(*)
PLANE_ANGLE_UNIT()
SI_UNIT($,.RADIAN.)
);
#34437=(
NAMED_UNIT(*)
SI_UNIT($,.STERADIAN.)
SOLID_ANGLE_UNIT()
);
#34448=SHAPE_DEFINITION_REPRESENTATION(#34476,#34547);
#34476=PRODUCT_DEFINITION_SHAPE('',$,#34576);
#34547=SHAPE_REPRESENTATION('',(#9399),#34415);
#34565=PRODUCT_DEFINITION_CONTEXT('part definition',#34651,'design');
#34576=PRODUCT_DEFINITION('Lower 60 mm clamp','Lower 60 mm clamp',#34604,
#34565);
#34604=PRODUCT_DEFINITION_FORMATION('',$,#34663);
#34651=APPLICATION_CONTEXT(
'Core Data for Automotive Mechanical Design Process');
#34652=PRODUCT_CONTEXT('part definition',#34651,'mechanical');
#34663=PRODUCT('Lower 60 mm clamp','Lower 60 mm clamp',
'Lower 60 mm clamp',(#34652));
#34751=COLOUR_RGB('Off White',0.89,0.88,0.83);
#34752=FILL_AREA_STYLE_COLOUR('',#34751);
#34753=FILL_AREA_STYLE('',(#34752));
#34754=SURFACE_STYLE_FILL_AREA(#34753);
#34755=SURFACE_SIDE_STYLE('',(#34754));
#34756=SURFACE_STYLE_USAGE(.BOTH.,#34755);
#34757=PRESENTATION_STYLE_ASSIGNMENT((#34756));
ENDSEC;
END-ISO-10303-21;
